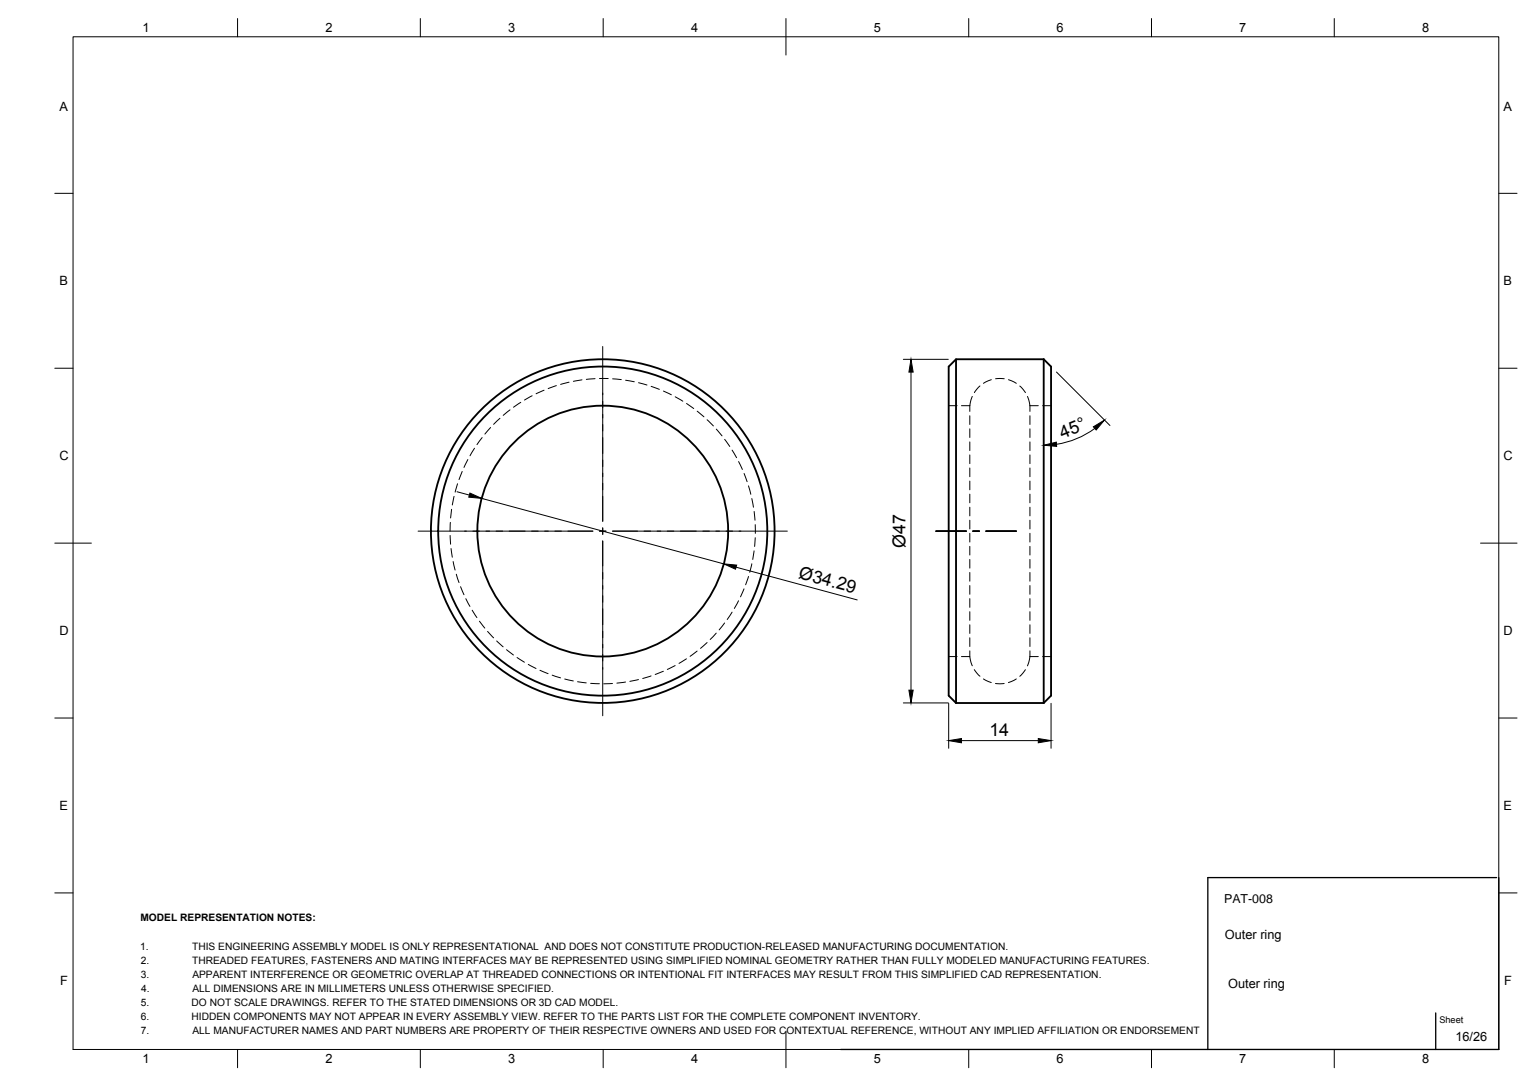
ISO-10303-21;
HEADER;
/* Generated by software containing ST-Developer
 * from STEP Tools, Inc. (www.steptools.com) 
 */

FILE_DESCRIPTION(
/* description */ ('Bearing housing with oil seal and end cap'),
/* implementation_level */ '2;1');

FILE_NAME(
/* name */ 'Outer ring.step',
/* time_stamp */ '2026-10-28T03:23:10-07:00',
/* author */ (''),
/* organization */ (''),
/* preprocessor_version */ 'ST-DEVELOPER v20.2',
/* originating_system */ 'Autodesk Translation Framework v15.17.0.0',
/* authorisation */ '');

FILE_SCHEMA (('AUTOMOTIVE_DESIGN { 1 0 10303 214 3 1 1 }'));
ENDSEC;

DATA;
#10=MECHANICAL_DESIGN_GEOMETRIC_PRESENTATION_REPRESENTATION('',(#268),#7871);
#203=CONICAL_SURFACE('',#4588,2.3,0.785398163397449);
#204=CONICAL_SURFACE('',#4592,2.3,0.785398163397449);
#216=TOROIDAL_SURFACE('',#4577,1.675,0.412776);
#226=SHAPE_REPRESENTATION_RELATIONSHIP('SRR','None',#7974,#247);
#247=ADVANCED_BREP_SHAPE_REPRESENTATION('',(#297),#7858);
#268=STYLED_ITEM('',(#8153),#297);
#297=MANIFOLD_SOLID_BREP('Body1',#4094);
#376=FACE_BOUND('',#980,.T.);
#377=FACE_BOUND('',#985,.T.);
#473=PLANE('',#4585);
#474=PLANE('',#4594);
#665=FACE_OUTER_BOUND('',#977,.T.);
#666=FACE_OUTER_BOUND('',#978,.T.);
#667=FACE_OUTER_BOUND('',#979,.T.);
#668=FACE_OUTER_BOUND('',#981,.T.);
#669=FACE_OUTER_BOUND('',#982,.T.);
#670=FACE_OUTER_BOUND('',#983,.T.);
#671=FACE_OUTER_BOUND('',#984,.T.);
#672=FACE_OUTER_BOUND('',#986,.T.);
#977=EDGE_LOOP('',(#3187,#3188,#3189,#3190,#3191,#3192));
#978=EDGE_LOOP('',(#3193,#3194,#3195,#3196,#3197));
#979=EDGE_LOOP('',(#3198));
#980=EDGE_LOOP('',(#3199));
#981=EDGE_LOOP('',(#3200,#3201,#3202,#3203));
#982=EDGE_LOOP('',(#3204,#3205,#3206,#3207));
#983=EDGE_LOOP('',(#3208,#3209,#3210,#3211));
#984=EDGE_LOOP('',(#3212));
#985=EDGE_LOOP('',(#3213));
#986=EDGE_LOOP('',(#3214,#3215,#3216,#3217,#3218));
#1266=LINE('',#6713,#1528);
#1267=LINE('',#6722,#1529);
#1268=LINE('',#6726,#1530);
#1269=LINE('',#6730,#1531);
#1270=LINE('',#6733,#1532);
#1528=VECTOR('',#5473,1.71469);
#1529=VECTOR('',#5484,2.3);
#1530=VECTOR('',#5489,2.35);
#1531=VECTOR('',#5494,2.3);
#1532=VECTOR('',#5499,1.71469);
#1774=CIRCLE('',#4578,1.71469);
#1775=CIRCLE('',#4579,1.71469);
#1776=CIRCLE('',#4580,0.412776);
#1777=CIRCLE('',#4581,1.71469);
#1778=CIRCLE('',#4582,1.71469);
#1779=CIRCLE('',#4584,1.71469);
#1780=CIRCLE('',#4586,2.25);
#1781=CIRCLE('',#4587,1.71469);
#1782=CIRCLE('',#4589,2.35);
#1783=CIRCLE('',#4591,2.35);
#1784=CIRCLE('',#4593,2.25);
#2037=VERTEX_POINT('',#6701);
#2038=VERTEX_POINT('',#6702);
#2039=VERTEX_POINT('',#6705);
#2040=VERTEX_POINT('',#6707);
#2041=VERTEX_POINT('',#6711);
#2042=VERTEX_POINT('',#6715);
#2043=VERTEX_POINT('',#6717);
#2044=VERTEX_POINT('',#6720);
#2045=VERTEX_POINT('',#6724);
#2046=VERTEX_POINT('',#6728);
#2457=EDGE_CURVE('',#2037,#2038,#1774,.T.);
#2458=EDGE_CURVE('',#2038,#2037,#1775,.T.);
#2459=EDGE_CURVE('',#2038,#2039,#1776,.T.);
#2460=EDGE_CURVE('',#2040,#2039,#1777,.T.);
#2461=EDGE_CURVE('',#2039,#2040,#1778,.T.);
#2462=EDGE_CURVE('',#2041,#2041,#1779,.T.);
#2463=EDGE_CURVE('',#2041,#2040,#1266,.T.);
#2464=EDGE_CURVE('',#2042,#2042,#1780,.T.);
#2465=EDGE_CURVE('',#2043,#2043,#1781,.T.);
#2466=EDGE_CURVE('',#2044,#2044,#1782,.T.);
#2467=EDGE_CURVE('',#2044,#2042,#1267,.T.);
#2468=EDGE_CURVE('',#2045,#2045,#1783,.T.);
#2469=EDGE_CURVE('',#2045,#2044,#1268,.T.);
#2470=EDGE_CURVE('',#2046,#2046,#1784,.T.);
#2471=EDGE_CURVE('',#2046,#2045,#1269,.T.);
#2472=EDGE_CURVE('',#2037,#2043,#1270,.T.);
#3187=ORIENTED_EDGE('',*,*,#2457,.F.);
#3188=ORIENTED_EDGE('',*,*,#2458,.F.);
#3189=ORIENTED_EDGE('',*,*,#2459,.T.);
#3190=ORIENTED_EDGE('',*,*,#2460,.F.);
#3191=ORIENTED_EDGE('',*,*,#2461,.F.);
#3192=ORIENTED_EDGE('',*,*,#2459,.F.);
#3193=ORIENTED_EDGE('',*,*,#2462,.T.);
#3194=ORIENTED_EDGE('',*,*,#2463,.T.);
#3195=ORIENTED_EDGE('',*,*,#2460,.T.);
#3196=ORIENTED_EDGE('',*,*,#2461,.T.);
#3197=ORIENTED_EDGE('',*,*,#2463,.F.);
#3198=ORIENTED_EDGE('',*,*,#2464,.F.);
#3199=ORIENTED_EDGE('',*,*,#2465,.T.);
#3200=ORIENTED_EDGE('',*,*,#2466,.F.);
#3201=ORIENTED_EDGE('',*,*,#2467,.T.);
#3202=ORIENTED_EDGE('',*,*,#2464,.T.);
#3203=ORIENTED_EDGE('',*,*,#2467,.F.);
#3204=ORIENTED_EDGE('',*,*,#2468,.F.);
#3205=ORIENTED_EDGE('',*,*,#2469,.T.);
#3206=ORIENTED_EDGE('',*,*,#2466,.T.);
#3207=ORIENTED_EDGE('',*,*,#2469,.F.);
#3208=ORIENTED_EDGE('',*,*,#2470,.F.);
#3209=ORIENTED_EDGE('',*,*,#2471,.T.);
#3210=ORIENTED_EDGE('',*,*,#2468,.T.);
#3211=ORIENTED_EDGE('',*,*,#2471,.F.);
#3212=ORIENTED_EDGE('',*,*,#2470,.T.);
#3213=ORIENTED_EDGE('',*,*,#2462,.F.);
#3214=ORIENTED_EDGE('',*,*,#2457,.T.);
#3215=ORIENTED_EDGE('',*,*,#2458,.T.);
#3216=ORIENTED_EDGE('',*,*,#2472,.T.);
#3217=ORIENTED_EDGE('',*,*,#2465,.F.);
#3218=ORIENTED_EDGE('',*,*,#2472,.F.);
#3804=CYLINDRICAL_SURFACE('',#4583,1.71469);
#3805=CYLINDRICAL_SURFACE('',#4590,2.35);
#3806=CYLINDRICAL_SURFACE('',#4595,1.71469);
#3947=ADVANCED_FACE('',(#665),#216,.F.);
#3948=ADVANCED_FACE('',(#666),#3804,.F.);
#3949=ADVANCED_FACE('',(#667,#376),#473,.T.);
#3950=ADVANCED_FACE('',(#668),#203,.T.);
#3951=ADVANCED_FACE('',(#669),#3805,.T.);
#3952=ADVANCED_FACE('',(#670),#204,.T.);
#3953=ADVANCED_FACE('',(#671,#377),#474,.T.);
#3954=ADVANCED_FACE('',(#672),#3806,.F.);
#4094=CLOSED_SHELL('',(#3947,#3948,#3949,#3950,#3951,#3952,#3953,#3954));
#4576=AXIS2_PLACEMENT_3D('',#6699,#5455,#5456);
#4577=AXIS2_PLACEMENT_3D('',#6700,#5457,#5458);
#4578=AXIS2_PLACEMENT_3D('',#6703,#5459,#5460);
#4579=AXIS2_PLACEMENT_3D('',#6704,#5461,#5462);
#4580=AXIS2_PLACEMENT_3D('',#6706,#5463,#5464);
#4581=AXIS2_PLACEMENT_3D('',#6708,#5465,#5466);
#4582=AXIS2_PLACEMENT_3D('',#6709,#5467,#5468);
#4583=AXIS2_PLACEMENT_3D('',#6710,#5469,#5470);
#4584=AXIS2_PLACEMENT_3D('',#6712,#5471,#5472);
#4585=AXIS2_PLACEMENT_3D('',#6714,#5474,#5475);
#4586=AXIS2_PLACEMENT_3D('',#6716,#5476,#5477);
#4587=AXIS2_PLACEMENT_3D('',#6718,#5478,#5479);
#4588=AXIS2_PLACEMENT_3D('',#6719,#5480,#5481);
#4589=AXIS2_PLACEMENT_3D('',#6721,#5482,#5483);
#4590=AXIS2_PLACEMENT_3D('',#6723,#5485,#5486);
#4591=AXIS2_PLACEMENT_3D('',#6725,#5487,#5488);
#4592=AXIS2_PLACEMENT_3D('',#6727,#5490,#5491);
#4593=AXIS2_PLACEMENT_3D('',#6729,#5492,#5493);
#4594=AXIS2_PLACEMENT_3D('',#6731,#5495,#5496);
#4595=AXIS2_PLACEMENT_3D('',#6732,#5497,#5498);
#5455=DIRECTION('axis',(0.,0.,1.));
#5456=DIRECTION('refdir',(1.,0.,0.));
#5457=DIRECTION('center_axis',(0.,-1.,0.));
#5458=DIRECTION('ref_axis',(0.,0.,-1.));
#5459=DIRECTION('center_axis',(0.,-1.,0.));
#5460=DIRECTION('ref_axis',(1.,0.,0.));
#5461=DIRECTION('center_axis',(0.,-1.,0.));
#5462=DIRECTION('ref_axis',(1.,0.,0.));
#5463=DIRECTION('center_axis',(1.,0.,1.22464679914735E-16));
#5464=DIRECTION('ref_axis',(-1.22464679914735E-16,0.,1.));
#5465=DIRECTION('center_axis',(0.,1.,0.));
#5466=DIRECTION('ref_axis',(1.,0.,0.));
#5467=DIRECTION('center_axis',(0.,1.,0.));
#5468=DIRECTION('ref_axis',(1.,0.,0.));
#5469=DIRECTION('center_axis',(0.,-1.,0.));
#5470=DIRECTION('ref_axis',(1.,0.,0.));
#5471=DIRECTION('center_axis',(0.,-1.,0.));
#5472=DIRECTION('ref_axis',(1.,0.,0.));
#5473=DIRECTION('',(0.,1.,0.));
#5474=DIRECTION('center_axis',(0.,1.,0.));
#5475=DIRECTION('ref_axis',(0.,0.,1.));
#5476=DIRECTION('center_axis',(0.,-1.,0.));
#5477=DIRECTION('ref_axis',(1.,0.,0.));
#5478=DIRECTION('center_axis',(0.,-1.,0.));
#5479=DIRECTION('ref_axis',(1.,0.,0.));
#5480=DIRECTION('center_axis',(0.,-1.,0.));
#5481=DIRECTION('ref_axis',(1.,0.,0.));
#5482=DIRECTION('center_axis',(0.,-1.,0.));
#5483=DIRECTION('ref_axis',(1.,0.,0.));
#5484=DIRECTION('',(0.707106781186548,0.707106781186547,8.65956056235494E-17));
#5485=DIRECTION('center_axis',(0.,-1.,0.));
#5486=DIRECTION('ref_axis',(1.,0.,0.));
#5487=DIRECTION('center_axis',(0.,-1.,0.));
#5488=DIRECTION('ref_axis',(1.,0.,0.));
#5489=DIRECTION('',(0.,1.,0.));
#5490=DIRECTION('center_axis',(0.,1.,0.));
#5491=DIRECTION('ref_axis',(1.,0.,0.));
#5492=DIRECTION('center_axis',(0.,-1.,0.));
#5493=DIRECTION('ref_axis',(1.,0.,0.));
#5494=DIRECTION('',(-0.707106781186548,0.707106781186547,-8.65956056235494E-17));
#5495=DIRECTION('center_axis',(0.,-1.,0.));
#5496=DIRECTION('ref_axis',(0.,0.,-1.));
#5497=DIRECTION('center_axis',(0.,-1.,0.));
#5498=DIRECTION('ref_axis',(1.,0.,0.));
#5499=DIRECTION('',(0.,1.,0.));
#6699=CARTESIAN_POINT('',(0.,0.,0.));
#6700=CARTESIAN_POINT('Origin',(0.,0.,0.));
#6701=CARTESIAN_POINT('',(-1.71469,0.410863395882378,-2.09988962002998E-16));
#6702=CARTESIAN_POINT('',(-2.09988962002998E-16,0.410863395882378,1.71469));
#6703=CARTESIAN_POINT('Origin',(0.,0.410863395882378,0.));
#6704=CARTESIAN_POINT('Origin',(0.,0.410863395882378,0.));
#6705=CARTESIAN_POINT('',(-2.09988962002998E-16,-0.410863395882378,1.71469));
#6706=CARTESIAN_POINT('Origin',(-2.05128338857182E-16,0.,1.675));
#6707=CARTESIAN_POINT('',(-1.71469,-0.410863395882378,2.09988962002998E-16));
#6708=CARTESIAN_POINT('Origin',(0.,-0.410863395882378,0.));
#6709=CARTESIAN_POINT('Origin',(0.,-0.410863395882378,0.));
#6710=CARTESIAN_POINT('Origin',(0.,0.,0.));
#6711=CARTESIAN_POINT('',(-1.71469,-0.7,-2.09988962002998E-16));
#6712=CARTESIAN_POINT('Origin',(0.,-0.7,0.));
#6713=CARTESIAN_POINT('',(-1.71469,0.,-2.09988962002998E-16));
#6714=CARTESIAN_POINT('Origin',(2.25,0.7,0.));
#6715=CARTESIAN_POINT('',(-2.25,0.7,-2.75545529808154E-16));
#6716=CARTESIAN_POINT('Origin',(0.,0.7,0.));
#6717=CARTESIAN_POINT('',(-1.71469,0.7,-2.09988962002998E-16));
#6718=CARTESIAN_POINT('Origin',(0.,0.7,0.));
#6719=CARTESIAN_POINT('Origin',(0.,0.65,0.));
#6720=CARTESIAN_POINT('',(-2.35,0.6,-2.87791997799628E-16));
#6721=CARTESIAN_POINT('Origin',(0.,0.6,0.));
#6722=CARTESIAN_POINT('',(-2.3,0.65,-2.81668763803891E-16));
#6723=CARTESIAN_POINT('Origin',(0.,0.,0.));
#6724=CARTESIAN_POINT('',(-2.35,-0.6,-2.87791997799628E-16));
#6725=CARTESIAN_POINT('Origin',(0.,-0.6,0.));
#6726=CARTESIAN_POINT('',(-2.35,0.,-2.87791997799628E-16));
#6727=CARTESIAN_POINT('Origin',(0.,-0.65,0.));
#6728=CARTESIAN_POINT('',(-2.25,-0.7,-2.75545529808154E-16));
#6729=CARTESIAN_POINT('Origin',(0.,-0.7,0.));
#6730=CARTESIAN_POINT('',(-2.3,-0.65,-2.81668763803891E-16));
#6731=CARTESIAN_POINT('Origin',(1.71469,-0.7,0.));
#6732=CARTESIAN_POINT('Origin',(0.,0.,0.));
#6733=CARTESIAN_POINT('',(-1.71469,0.,-2.09988962002998E-16));
#7832=UNCERTAINTY_MEASURE_WITH_UNIT(LENGTH_MEASURE(0.001),#7872,
'DISTANCE_ACCURACY_VALUE',
'Maximum model space distance between geometric entities at asserted c
onnectivities');
#7845=UNCERTAINTY_MEASURE_WITH_UNIT(LENGTH_MEASURE(0.001),#7872,
'DISTANCE_ACCURACY_VALUE',
'Maximum model space distance between geometric entities at asserted c
onnectivities');
#7858=(
GEOMETRIC_REPRESENTATION_CONTEXT(3)
GLOBAL_UNCERTAINTY_ASSIGNED_CONTEXT((#7832))
GLOBAL_UNIT_ASSIGNED_CONTEXT((#7872,#7874,#7875))
REPRESENTATION_CONTEXT('','3D')
);
#7871=(
GEOMETRIC_REPRESENTATION_CONTEXT(3)
GLOBAL_UNCERTAINTY_ASSIGNED_CONTEXT((#7845))
GLOBAL_UNIT_ASSIGNED_CONTEXT((#7872,#7874,#7875))
REPRESENTATION_CONTEXT('','3D')
);
#7872=(
LENGTH_UNIT()
NAMED_UNIT(*)
SI_UNIT(.CENTI.,.METRE.)
);
#7874=(
NAMED_UNIT(*)
PLANE_ANGLE_UNIT()
SI_UNIT($,.RADIAN.)
);
#7875=(
NAMED_UNIT(*)
SI_UNIT($,.STERADIAN.)
SOLID_ANGLE_UNIT()
);
#7888=SHAPE_DEFINITION_REPRESENTATION(#7913,#7974);
#7913=PRODUCT_DEFINITION_SHAPE('',$,#8000);
#7974=SHAPE_REPRESENTATION('',(#4576),#7858);
#7987=PRODUCT_DEFINITION_CONTEXT('part definition',#8064,'design');
#8000=PRODUCT_DEFINITION('Outer ring','Outer ring',#8025,#7987);
#8025=PRODUCT_DEFINITION_FORMATION('',$,#8078);
#8064=APPLICATION_CONTEXT(
'Core Data for Automotive Mechanical Design Process');
#8065=PRODUCT_CONTEXT('part definition',#8064,'mechanical');
#8078=PRODUCT('Outer ring','Outer ring','Outer ring',(#8065));
#8147=COLOUR_RGB('Grey',0.48,0.52,0.57);
#8148=FILL_AREA_STYLE_COLOUR('',#8147);
#8149=FILL_AREA_STYLE('',(#8148));
#8150=SURFACE_STYLE_FILL_AREA(#8149);
#8151=SURFACE_SIDE_STYLE('',(#8150));
#8152=SURFACE_STYLE_USAGE(.BOTH.,#8151);
#8153=PRESENTATION_STYLE_ASSIGNMENT((#8152));
ENDSEC;
END-ISO-10303-21;
